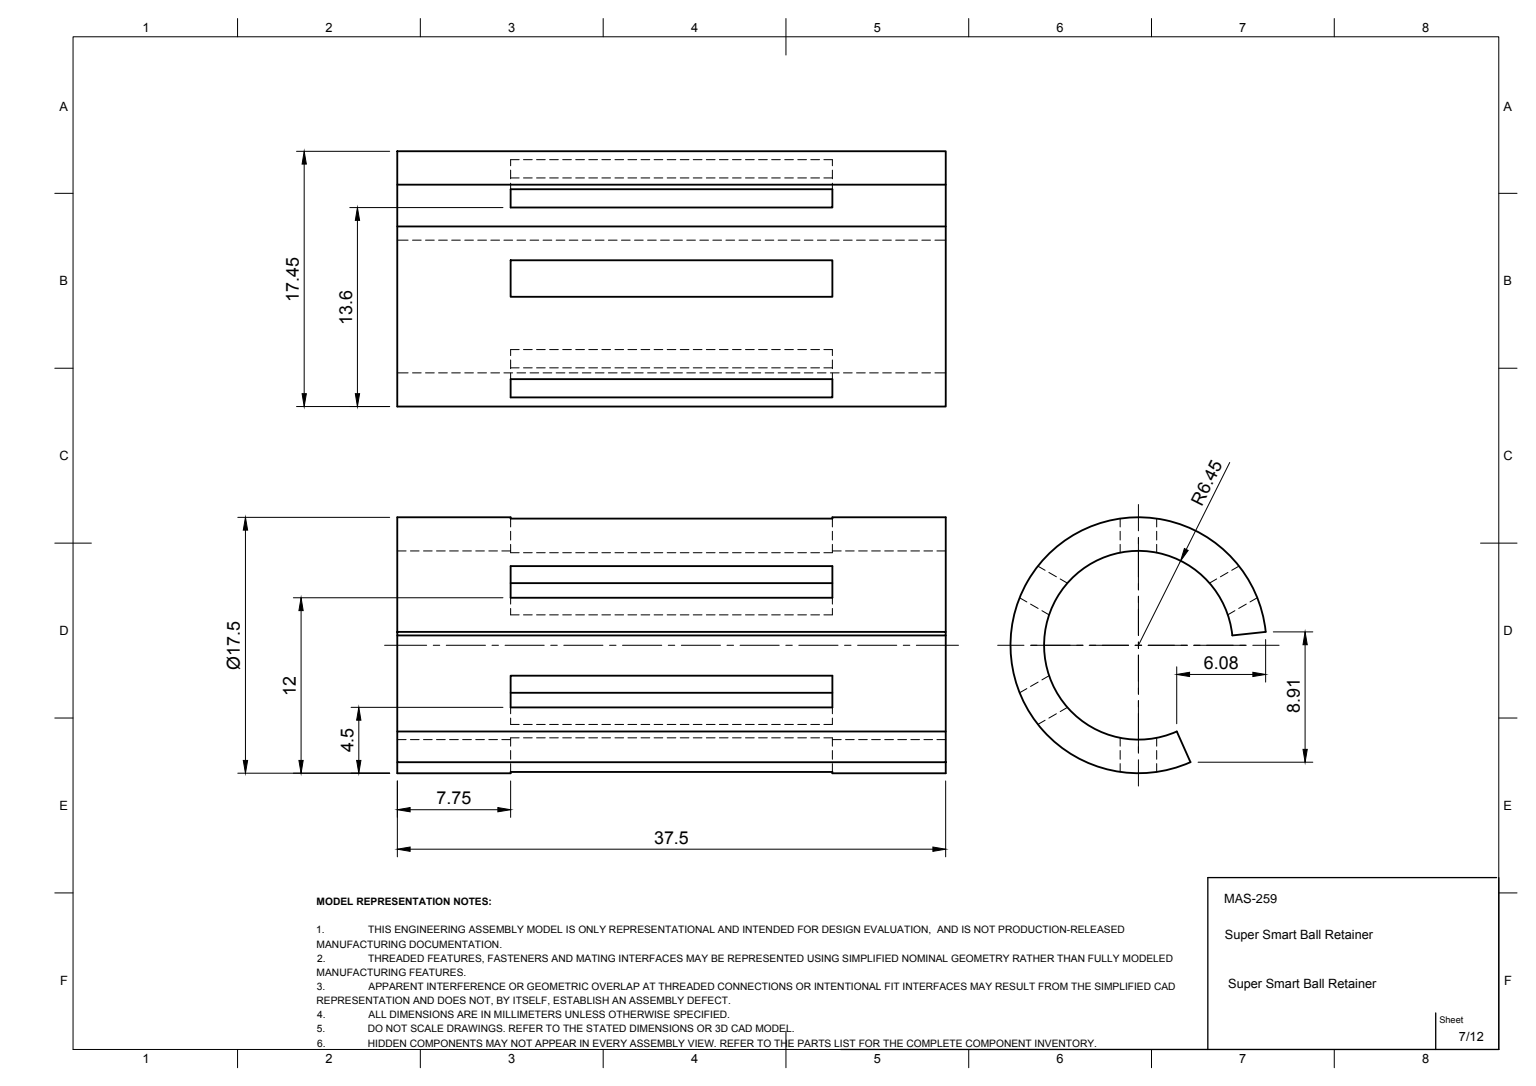
ISO-10303-21;
HEADER;
/* Generated by software containing ST-Developer
 * from STEP Tools, Inc. (www.steptools.com) 
 */

FILE_DESCRIPTION(
/* description */ (''),
/* implementation_level */ '2;1');

FILE_NAME(
/* name */ 'Super Smart Ball Retainer.step',
/* time_stamp */ '2026-10-15T13:30:17-07:00',
/* author */ (''),
/* organization */ (''),
/* preprocessor_version */ 'ST-DEVELOPER v20.2',
/* originating_system */ 'Autodesk Translation Framework v15.15.0.0',
/* authorisation */ '');

FILE_SCHEMA (('AUTOMOTIVE_DESIGN { 1 0 10303 214 3 1 1 }'));
ENDSEC;

DATA;
#10=MECHANICAL_DESIGN_GEOMETRIC_PRESENTATION_REPRESENTATION('',(#1038),#71795);
#1018=SHAPE_REPRESENTATION_RELATIONSHIP('SRR','None',#72022,#1028);
#1028=ADVANCED_BREP_SHAPE_REPRESENTATION('',(#1048),#71790);
#1038=STYLED_ITEM('',(#72081),#1048);
#1048=MANIFOLD_SOLID_BREP('Body1',#13640);
#1549=FACE_BOUND('',#2923,.T.);
#1550=FACE_BOUND('',#2924,.T.);
#1551=FACE_BOUND('',#2925,.T.);
#1552=FACE_BOUND('',#2926,.T.);
#1553=FACE_BOUND('',#2927,.T.);
#1554=FACE_BOUND('',#2929,.T.);
#1555=FACE_BOUND('',#2930,.T.);
#1556=FACE_BOUND('',#2931,.T.);
#1557=FACE_BOUND('',#2932,.T.);
#1558=FACE_BOUND('',#2933,.T.);
#1628=PLANE('',#14061);
#1629=PLANE('',#14062);
#1630=PLANE('',#14065);
#1631=PLANE('',#14066);
#1632=PLANE('',#14069);
#1633=PLANE('',#14070);
#1634=PLANE('',#14073);
#1635=PLANE('',#14074);
#1636=PLANE('',#14077);
#1637=PLANE('',#14078);
#1638=PLANE('',#14081);
#1639=PLANE('',#14082);
#1640=PLANE('',#14085);
#1641=PLANE('',#14086);
#1642=PLANE('',#14089);
#1643=PLANE('',#14090);
#1644=PLANE('',#14093);
#1645=PLANE('',#14094);
#1646=PLANE('',#14097);
#1647=PLANE('',#14098);
#1648=PLANE('',#14101);
#1649=PLANE('',#14102);
#1650=PLANE('',#14103);
#1651=PLANE('',#14110);
#2186=FACE_OUTER_BOUND('',#2899,.T.);
#2187=FACE_OUTER_BOUND('',#2900,.T.);
#2188=FACE_OUTER_BOUND('',#2901,.T.);
#2189=FACE_OUTER_BOUND('',#2902,.T.);
#2190=FACE_OUTER_BOUND('',#2903,.T.);
#2191=FACE_OUTER_BOUND('',#2904,.T.);
#2192=FACE_OUTER_BOUND('',#2905,.T.);
#2193=FACE_OUTER_BOUND('',#2906,.T.);
#2194=FACE_OUTER_BOUND('',#2907,.T.);
#2195=FACE_OUTER_BOUND('',#2908,.T.);
#2196=FACE_OUTER_BOUND('',#2909,.T.);
#2197=FACE_OUTER_BOUND('',#2910,.T.);
#2198=FACE_OUTER_BOUND('',#2911,.T.);
#2199=FACE_OUTER_BOUND('',#2912,.T.);
#2200=FACE_OUTER_BOUND('',#2913,.T.);
#2201=FACE_OUTER_BOUND('',#2914,.T.);
#2202=FACE_OUTER_BOUND('',#2915,.T.);
#2203=FACE_OUTER_BOUND('',#2916,.T.);
#2204=FACE_OUTER_BOUND('',#2917,.T.);
#2205=FACE_OUTER_BOUND('',#2918,.T.);
#2206=FACE_OUTER_BOUND('',#2919,.T.);
#2207=FACE_OUTER_BOUND('',#2920,.T.);
#2208=FACE_OUTER_BOUND('',#2921,.T.);
#2209=FACE_OUTER_BOUND('',#2922,.T.);
#2210=FACE_OUTER_BOUND('',#2928,.T.);
#2211=FACE_OUTER_BOUND('',#2934,.T.);
#2899=EDGE_LOOP('',(#9713,#9714,#9715,#9716));
#2900=EDGE_LOOP('',(#9717,#9718,#9719,#9720));
#2901=EDGE_LOOP('',(#9721,#9722,#9723,#9724));
#2902=EDGE_LOOP('',(#9725,#9726,#9727,#9728));
#2903=EDGE_LOOP('',(#9729,#9730,#9731,#9732));
#2904=EDGE_LOOP('',(#9733,#9734,#9735,#9736));
#2905=EDGE_LOOP('',(#9737,#9738,#9739,#9740));
#2906=EDGE_LOOP('',(#9741,#9742,#9743,#9744));
#2907=EDGE_LOOP('',(#9745,#9746,#9747,#9748));
#2908=EDGE_LOOP('',(#9749,#9750,#9751,#9752));
#2909=EDGE_LOOP('',(#9753,#9754,#9755,#9756));
#2910=EDGE_LOOP('',(#9757,#9758,#9759,#9760));
#2911=EDGE_LOOP('',(#9761,#9762,#9763,#9764));
#2912=EDGE_LOOP('',(#9765,#9766,#9767,#9768));
#2913=EDGE_LOOP('',(#9769,#9770,#9771,#9772));
#2914=EDGE_LOOP('',(#9773,#9774,#9775,#9776));
#2915=EDGE_LOOP('',(#9777,#9778,#9779,#9780));
#2916=EDGE_LOOP('',(#9781,#9782,#9783,#9784));
#2917=EDGE_LOOP('',(#9785,#9786,#9787,#9788));
#2918=EDGE_LOOP('',(#9789,#9790,#9791,#9792));
#2919=EDGE_LOOP('',(#9793,#9794,#9795,#9796));
#2920=EDGE_LOOP('',(#9797,#9798,#9799,#9800));
#2921=EDGE_LOOP('',(#9801,#9802,#9803,#9804));
#2922=EDGE_LOOP('',(#9805,#9806,#9807,#9808));
#2923=EDGE_LOOP('',(#9809,#9810,#9811,#9812));
#2924=EDGE_LOOP('',(#9813,#9814,#9815,#9816));
#2925=EDGE_LOOP('',(#9817,#9818,#9819,#9820));
#2926=EDGE_LOOP('',(#9821,#9822,#9823,#9824));
#2927=EDGE_LOOP('',(#9825,#9826,#9827,#9828));
#2928=EDGE_LOOP('',(#9829,#9830,#9831,#9832));
#2929=EDGE_LOOP('',(#9833,#9834,#9835,#9836));
#2930=EDGE_LOOP('',(#9837,#9838,#9839,#9840));
#2931=EDGE_LOOP('',(#9841,#9842,#9843,#9844));
#2932=EDGE_LOOP('',(#9845,#9846,#9847,#9848));
#2933=EDGE_LOOP('',(#9849,#9850,#9851,#9852));
#2934=EDGE_LOOP('',(#9853,#9854,#9855,#9856));
#3537=CIRCLE('',#14063,8.75);
#3538=CIRCLE('',#14064,6.45);
#3539=CIRCLE('',#14067,8.75);
#3540=CIRCLE('',#14068,6.45);
#3541=CIRCLE('',#14071,8.75);
#3542=CIRCLE('',#14072,6.45);
#3543=CIRCLE('',#14075,8.75);
#3544=CIRCLE('',#14076,6.45);
#3545=CIRCLE('',#14079,8.75);
#3546=CIRCLE('',#14080,6.45);
#3547=CIRCLE('',#14083,8.75);
#3548=CIRCLE('',#14084,6.45);
#3549=CIRCLE('',#14087,8.75);
#3550=CIRCLE('',#14088,6.45);
#3551=CIRCLE('',#14091,8.75);
#3552=CIRCLE('',#14092,6.45);
#3553=CIRCLE('',#14095,8.75);
#3554=CIRCLE('',#14096,6.45);
#3555=CIRCLE('',#14099,8.75);
#3556=CIRCLE('',#14100,6.45);
#3557=CIRCLE('',#14104,6.45);
#3558=CIRCLE('',#14105,8.75);
#3559=CIRCLE('',#14107,8.75);
#3560=CIRCLE('',#14109,6.45);
#4035=LINE('',#19743,#4946);
#4036=LINE('',#19745,#4947);
#4037=LINE('',#19747,#4948);
#4038=LINE('',#19748,#4949);
#4039=LINE('',#19754,#4950);
#4040=LINE('',#19757,#4951);
#4041=LINE('',#19759,#4952);
#4042=LINE('',#19760,#4953);
#4043=LINE('',#19767,#4954);
#4044=LINE('',#19769,#4955);
#4045=LINE('',#19771,#4956);
#4046=LINE('',#19772,#4957);
#4047=LINE('',#19778,#4958);
#4048=LINE('',#19781,#4959);
#4049=LINE('',#19783,#4960);
#4050=LINE('',#19784,#4961);
#4051=LINE('',#19791,#4962);
#4052=LINE('',#19793,#4963);
#4053=LINE('',#19795,#4964);
#4054=LINE('',#19796,#4965);
#4055=LINE('',#19802,#4966);
#4056=LINE('',#19805,#4967);
#4057=LINE('',#19807,#4968);
#4058=LINE('',#19808,#4969);
#4059=LINE('',#19815,#4970);
#4060=LINE('',#19817,#4971);
#4061=LINE('',#19819,#4972);
#4062=LINE('',#19820,#4973);
#4063=LINE('',#19826,#4974);
#4064=LINE('',#19829,#4975);
#4065=LINE('',#19831,#4976);
#4066=LINE('',#19832,#4977);
#4067=LINE('',#19839,#4978);
#4068=LINE('',#19841,#4979);
#4069=LINE('',#19843,#4980);
#4070=LINE('',#19844,#4981);
#4071=LINE('',#19850,#4982);
#4072=LINE('',#19853,#4983);
#4073=LINE('',#19855,#4984);
#4074=LINE('',#19856,#4985);
#4075=LINE('',#19863,#4986);
#4076=LINE('',#19865,#4987);
#4077=LINE('',#19867,#4988);
#4078=LINE('',#19868,#4989);
#4079=LINE('',#19872,#4990);
#4080=LINE('',#19874,#4991);
#4081=LINE('',#19876,#4992);
#4082=LINE('',#19877,#4993);
#4946=VECTOR('',#15852,10.);
#4947=VECTOR('',#15853,10.);
#4948=VECTOR('',#15854,10.);
#4949=VECTOR('',#15855,10.);
#4950=VECTOR('',#15862,10.);
#4951=VECTOR('',#15865,10.);
#4952=VECTOR('',#15866,10.);
#4953=VECTOR('',#15867,10.);
#4954=VECTOR('',#15876,10.);
#4955=VECTOR('',#15877,10.);
#4956=VECTOR('',#15878,10.);
#4957=VECTOR('',#15879,10.);
#4958=VECTOR('',#15886,10.);
#4959=VECTOR('',#15889,10.);
#4960=VECTOR('',#15890,10.);
#4961=VECTOR('',#15891,10.);
#4962=VECTOR('',#15900,10.);
#4963=VECTOR('',#15901,10.);
#4964=VECTOR('',#15902,10.);
#4965=VECTOR('',#15903,10.);
#4966=VECTOR('',#15910,9.99999999999999);
#4967=VECTOR('',#15913,10.);
#4968=VECTOR('',#15914,10.);
#4969=VECTOR('',#15915,9.99999999999999);
#4970=VECTOR('',#15924,10.);
#4971=VECTOR('',#15925,9.99999999999999);
#4972=VECTOR('',#15926,10.);
#4973=VECTOR('',#15927,9.99999999999999);
#4974=VECTOR('',#15934,10.);
#4975=VECTOR('',#15937,10.);
#4976=VECTOR('',#15938,10.);
#4977=VECTOR('',#15939,10.);
#4978=VECTOR('',#15948,10.);
#4979=VECTOR('',#15949,9.99999999999999);
#4980=VECTOR('',#15950,10.);
#4981=VECTOR('',#15951,9.99999999999999);
#4982=VECTOR('',#15958,10.);
#4983=VECTOR('',#15961,10.);
#4984=VECTOR('',#15962,10.);
#4985=VECTOR('',#15963,10.);
#4986=VECTOR('',#15972,10.);
#4987=VECTOR('',#15973,10.);
#4988=VECTOR('',#15974,10.);
#4989=VECTOR('',#15975,10.);
#4990=VECTOR('',#15978,10.);
#4991=VECTOR('',#15979,10.);
#4992=VECTOR('',#15980,10.);
#4993=VECTOR('',#15981,10.);
#5916=VERTEX_POINT('',#19741);
#5917=VERTEX_POINT('',#19742);
#5918=VERTEX_POINT('',#19744);
#5919=VERTEX_POINT('',#19746);
#5920=VERTEX_POINT('',#19750);
#5921=VERTEX_POINT('',#19752);
#5922=VERTEX_POINT('',#19756);
#5923=VERTEX_POINT('',#19758);
#5924=VERTEX_POINT('',#19765);
#5925=VERTEX_POINT('',#19766);
#5926=VERTEX_POINT('',#19768);
#5927=VERTEX_POINT('',#19770);
#5928=VERTEX_POINT('',#19774);
#5929=VERTEX_POINT('',#19776);
#5930=VERTEX_POINT('',#19780);
#5931=VERTEX_POINT('',#19782);
#5932=VERTEX_POINT('',#19789);
#5933=VERTEX_POINT('',#19790);
#5934=VERTEX_POINT('',#19792);
#5935=VERTEX_POINT('',#19794);
#5936=VERTEX_POINT('',#19798);
#5937=VERTEX_POINT('',#19800);
#5938=VERTEX_POINT('',#19804);
#5939=VERTEX_POINT('',#19806);
#5940=VERTEX_POINT('',#19813);
#5941=VERTEX_POINT('',#19814);
#5942=VERTEX_POINT('',#19816);
#5943=VERTEX_POINT('',#19818);
#5944=VERTEX_POINT('',#19822);
#5945=VERTEX_POINT('',#19824);
#5946=VERTEX_POINT('',#19828);
#5947=VERTEX_POINT('',#19830);
#5948=VERTEX_POINT('',#19837);
#5949=VERTEX_POINT('',#19838);
#5950=VERTEX_POINT('',#19840);
#5951=VERTEX_POINT('',#19842);
#5952=VERTEX_POINT('',#19846);
#5953=VERTEX_POINT('',#19848);
#5954=VERTEX_POINT('',#19852);
#5955=VERTEX_POINT('',#19854);
#5956=VERTEX_POINT('',#19861);
#5957=VERTEX_POINT('',#19862);
#5958=VERTEX_POINT('',#19864);
#5959=VERTEX_POINT('',#19866);
#5960=VERTEX_POINT('',#19870);
#5961=VERTEX_POINT('',#19871);
#5962=VERTEX_POINT('',#19873);
#5963=VERTEX_POINT('',#19875);
#7391=EDGE_CURVE('',#5916,#5917,#4035,.T.);
#7392=EDGE_CURVE('',#5916,#5918,#4036,.T.);
#7393=EDGE_CURVE('',#5919,#5918,#4037,.T.);
#7394=EDGE_CURVE('',#5919,#5917,#4038,.T.);
#7395=EDGE_CURVE('',#5917,#5920,#3537,.T.);
#7396=EDGE_CURVE('',#5921,#5919,#3538,.T.);
#7397=EDGE_CURVE('',#5920,#5921,#4039,.T.);
#7398=EDGE_CURVE('',#5920,#5922,#4040,.T.);
#7399=EDGE_CURVE('',#5923,#5921,#4041,.T.);
#7400=EDGE_CURVE('',#5923,#5922,#4042,.T.);
#7401=EDGE_CURVE('',#5922,#5916,#3539,.T.);
#7402=EDGE_CURVE('',#5918,#5923,#3540,.T.);
#7403=EDGE_CURVE('',#5924,#5925,#4043,.T.);
#7404=EDGE_CURVE('',#5924,#5926,#4044,.T.);
#7405=EDGE_CURVE('',#5927,#5926,#4045,.T.);
#7406=EDGE_CURVE('',#5927,#5925,#4046,.T.);
#7407=EDGE_CURVE('',#5925,#5928,#3541,.T.);
#7408=EDGE_CURVE('',#5929,#5927,#3542,.T.);
#7409=EDGE_CURVE('',#5928,#5929,#4047,.T.);
#7410=EDGE_CURVE('',#5928,#5930,#4048,.T.);
#7411=EDGE_CURVE('',#5931,#5929,#4049,.T.);
#7412=EDGE_CURVE('',#5931,#5930,#4050,.T.);
#7413=EDGE_CURVE('',#5930,#5924,#3543,.T.);
#7414=EDGE_CURVE('',#5926,#5931,#3544,.T.);
#7415=EDGE_CURVE('',#5932,#5933,#4051,.T.);
#7416=EDGE_CURVE('',#5932,#5934,#4052,.T.);
#7417=EDGE_CURVE('',#5935,#5934,#4053,.T.);
#7418=EDGE_CURVE('',#5935,#5933,#4054,.T.);
#7419=EDGE_CURVE('',#5933,#5936,#3545,.T.);
#7420=EDGE_CURVE('',#5937,#5935,#3546,.T.);
#7421=EDGE_CURVE('',#5936,#5937,#4055,.T.);
#7422=EDGE_CURVE('',#5936,#5938,#4056,.T.);
#7423=EDGE_CURVE('',#5939,#5937,#4057,.T.);
#7424=EDGE_CURVE('',#5939,#5938,#4058,.T.);
#7425=EDGE_CURVE('',#5938,#5932,#3547,.T.);
#7426=EDGE_CURVE('',#5934,#5939,#3548,.T.);
#7427=EDGE_CURVE('',#5940,#5941,#4059,.T.);
#7428=EDGE_CURVE('',#5940,#5942,#4060,.T.);
#7429=EDGE_CURVE('',#5943,#5942,#4061,.T.);
#7430=EDGE_CURVE('',#5943,#5941,#4062,.T.);
#7431=EDGE_CURVE('',#5941,#5944,#3549,.T.);
#7432=EDGE_CURVE('',#5945,#5943,#3550,.T.);
#7433=EDGE_CURVE('',#5944,#5945,#4063,.T.);
#7434=EDGE_CURVE('',#5944,#5946,#4064,.T.);
#7435=EDGE_CURVE('',#5947,#5945,#4065,.T.);
#7436=EDGE_CURVE('',#5947,#5946,#4066,.T.);
#7437=EDGE_CURVE('',#5946,#5940,#3551,.T.);
#7438=EDGE_CURVE('',#5942,#5947,#3552,.T.);
#7439=EDGE_CURVE('',#5948,#5949,#4067,.T.);
#7440=EDGE_CURVE('',#5948,#5950,#4068,.T.);
#7441=EDGE_CURVE('',#5951,#5950,#4069,.T.);
#7442=EDGE_CURVE('',#5951,#5949,#4070,.T.);
#7443=EDGE_CURVE('',#5949,#5952,#3553,.T.);
#7444=EDGE_CURVE('',#5953,#5951,#3554,.T.);
#7445=EDGE_CURVE('',#5952,#5953,#4071,.T.);
#7446=EDGE_CURVE('',#5952,#5954,#4072,.T.);
#7447=EDGE_CURVE('',#5955,#5953,#4073,.T.);
#7448=EDGE_CURVE('',#5955,#5954,#4074,.T.);
#7449=EDGE_CURVE('',#5954,#5948,#3555,.T.);
#7450=EDGE_CURVE('',#5950,#5955,#3556,.T.);
#7451=EDGE_CURVE('',#5956,#5957,#4075,.T.);
#7452=EDGE_CURVE('',#5958,#5956,#4076,.T.);
#7453=EDGE_CURVE('',#5959,#5958,#4077,.T.);
#7454=EDGE_CURVE('',#5957,#5959,#4078,.T.);
#7455=EDGE_CURVE('',#5960,#5961,#4079,.T.);
#7456=EDGE_CURVE('',#5962,#5960,#4080,.T.);
#7457=EDGE_CURVE('',#5963,#5962,#4081,.T.);
#7458=EDGE_CURVE('',#5961,#5963,#4082,.T.);
#7459=EDGE_CURVE('',#5961,#5956,#3557,.T.);
#7460=EDGE_CURVE('',#5963,#5958,#3558,.T.);
#7461=EDGE_CURVE('',#5962,#5959,#3559,.T.);
#7462=EDGE_CURVE('',#5960,#5957,#3560,.T.);
#9713=ORIENTED_EDGE('',*,*,#7391,.F.);
#9714=ORIENTED_EDGE('',*,*,#7392,.T.);
#9715=ORIENTED_EDGE('',*,*,#7393,.F.);
#9716=ORIENTED_EDGE('',*,*,#7394,.T.);
#9717=ORIENTED_EDGE('',*,*,#7395,.F.);
#9718=ORIENTED_EDGE('',*,*,#7394,.F.);
#9719=ORIENTED_EDGE('',*,*,#7396,.F.);
#9720=ORIENTED_EDGE('',*,*,#7397,.F.);
#9721=ORIENTED_EDGE('',*,*,#7398,.F.);
#9722=ORIENTED_EDGE('',*,*,#7397,.T.);
#9723=ORIENTED_EDGE('',*,*,#7399,.F.);
#9724=ORIENTED_EDGE('',*,*,#7400,.T.);
#9725=ORIENTED_EDGE('',*,*,#7401,.F.);
#9726=ORIENTED_EDGE('',*,*,#7400,.F.);
#9727=ORIENTED_EDGE('',*,*,#7402,.F.);
#9728=ORIENTED_EDGE('',*,*,#7392,.F.);
#9729=ORIENTED_EDGE('',*,*,#7403,.F.);
#9730=ORIENTED_EDGE('',*,*,#7404,.T.);
#9731=ORIENTED_EDGE('',*,*,#7405,.F.);
#9732=ORIENTED_EDGE('',*,*,#7406,.T.);
#9733=ORIENTED_EDGE('',*,*,#7407,.F.);
#9734=ORIENTED_EDGE('',*,*,#7406,.F.);
#9735=ORIENTED_EDGE('',*,*,#7408,.F.);
#9736=ORIENTED_EDGE('',*,*,#7409,.F.);
#9737=ORIENTED_EDGE('',*,*,#7410,.F.);
#9738=ORIENTED_EDGE('',*,*,#7409,.T.);
#9739=ORIENTED_EDGE('',*,*,#7411,.F.);
#9740=ORIENTED_EDGE('',*,*,#7412,.T.);
#9741=ORIENTED_EDGE('',*,*,#7413,.F.);
#9742=ORIENTED_EDGE('',*,*,#7412,.F.);
#9743=ORIENTED_EDGE('',*,*,#7414,.F.);
#9744=ORIENTED_EDGE('',*,*,#7404,.F.);
#9745=ORIENTED_EDGE('',*,*,#7415,.F.);
#9746=ORIENTED_EDGE('',*,*,#7416,.T.);
#9747=ORIENTED_EDGE('',*,*,#7417,.F.);
#9748=ORIENTED_EDGE('',*,*,#7418,.T.);
#9749=ORIENTED_EDGE('',*,*,#7419,.F.);
#9750=ORIENTED_EDGE('',*,*,#7418,.F.);
#9751=ORIENTED_EDGE('',*,*,#7420,.F.);
#9752=ORIENTED_EDGE('',*,*,#7421,.F.);
#9753=ORIENTED_EDGE('',*,*,#7422,.F.);
#9754=ORIENTED_EDGE('',*,*,#7421,.T.);
#9755=ORIENTED_EDGE('',*,*,#7423,.F.);
#9756=ORIENTED_EDGE('',*,*,#7424,.T.);
#9757=ORIENTED_EDGE('',*,*,#7425,.F.);
#9758=ORIENTED_EDGE('',*,*,#7424,.F.);
#9759=ORIENTED_EDGE('',*,*,#7426,.F.);
#9760=ORIENTED_EDGE('',*,*,#7416,.F.);
#9761=ORIENTED_EDGE('',*,*,#7427,.F.);
#9762=ORIENTED_EDGE('',*,*,#7428,.T.);
#9763=ORIENTED_EDGE('',*,*,#7429,.F.);
#9764=ORIENTED_EDGE('',*,*,#7430,.T.);
#9765=ORIENTED_EDGE('',*,*,#7431,.F.);
#9766=ORIENTED_EDGE('',*,*,#7430,.F.);
#9767=ORIENTED_EDGE('',*,*,#7432,.F.);
#9768=ORIENTED_EDGE('',*,*,#7433,.F.);
#9769=ORIENTED_EDGE('',*,*,#7434,.F.);
#9770=ORIENTED_EDGE('',*,*,#7433,.T.);
#9771=ORIENTED_EDGE('',*,*,#7435,.F.);
#9772=ORIENTED_EDGE('',*,*,#7436,.T.);
#9773=ORIENTED_EDGE('',*,*,#7437,.F.);
#9774=ORIENTED_EDGE('',*,*,#7436,.F.);
#9775=ORIENTED_EDGE('',*,*,#7438,.F.);
#9776=ORIENTED_EDGE('',*,*,#7428,.F.);
#9777=ORIENTED_EDGE('',*,*,#7439,.F.);
#9778=ORIENTED_EDGE('',*,*,#7440,.T.);
#9779=ORIENTED_EDGE('',*,*,#7441,.F.);
#9780=ORIENTED_EDGE('',*,*,#7442,.T.);
#9781=ORIENTED_EDGE('',*,*,#7443,.F.);
#9782=ORIENTED_EDGE('',*,*,#7442,.F.);
#9783=ORIENTED_EDGE('',*,*,#7444,.F.);
#9784=ORIENTED_EDGE('',*,*,#7445,.F.);
#9785=ORIENTED_EDGE('',*,*,#7446,.F.);
#9786=ORIENTED_EDGE('',*,*,#7445,.T.);
#9787=ORIENTED_EDGE('',*,*,#7447,.F.);
#9788=ORIENTED_EDGE('',*,*,#7448,.T.);
#9789=ORIENTED_EDGE('',*,*,#7449,.F.);
#9790=ORIENTED_EDGE('',*,*,#7448,.F.);
#9791=ORIENTED_EDGE('',*,*,#7450,.F.);
#9792=ORIENTED_EDGE('',*,*,#7440,.F.);
#9793=ORIENTED_EDGE('',*,*,#7451,.F.);
#9794=ORIENTED_EDGE('',*,*,#7452,.F.);
#9795=ORIENTED_EDGE('',*,*,#7453,.F.);
#9796=ORIENTED_EDGE('',*,*,#7454,.F.);
#9797=ORIENTED_EDGE('',*,*,#7455,.F.);
#9798=ORIENTED_EDGE('',*,*,#7456,.F.);
#9799=ORIENTED_EDGE('',*,*,#7457,.F.);
#9800=ORIENTED_EDGE('',*,*,#7458,.F.);
#9801=ORIENTED_EDGE('',*,*,#7452,.T.);
#9802=ORIENTED_EDGE('',*,*,#7459,.F.);
#9803=ORIENTED_EDGE('',*,*,#7458,.T.);
#9804=ORIENTED_EDGE('',*,*,#7460,.T.);
#9805=ORIENTED_EDGE('',*,*,#7453,.T.);
#9806=ORIENTED_EDGE('',*,*,#7460,.F.);
#9807=ORIENTED_EDGE('',*,*,#7457,.T.);
#9808=ORIENTED_EDGE('',*,*,#7461,.T.);
#9809=ORIENTED_EDGE('',*,*,#7398,.T.);
#9810=ORIENTED_EDGE('',*,*,#7401,.T.);
#9811=ORIENTED_EDGE('',*,*,#7391,.T.);
#9812=ORIENTED_EDGE('',*,*,#7395,.T.);
#9813=ORIENTED_EDGE('',*,*,#7410,.T.);
#9814=ORIENTED_EDGE('',*,*,#7413,.T.);
#9815=ORIENTED_EDGE('',*,*,#7403,.T.);
#9816=ORIENTED_EDGE('',*,*,#7407,.T.);
#9817=ORIENTED_EDGE('',*,*,#7422,.T.);
#9818=ORIENTED_EDGE('',*,*,#7425,.T.);
#9819=ORIENTED_EDGE('',*,*,#7415,.T.);
#9820=ORIENTED_EDGE('',*,*,#7419,.T.);
#9821=ORIENTED_EDGE('',*,*,#7434,.T.);
#9822=ORIENTED_EDGE('',*,*,#7437,.T.);
#9823=ORIENTED_EDGE('',*,*,#7427,.T.);
#9824=ORIENTED_EDGE('',*,*,#7431,.T.);
#9825=ORIENTED_EDGE('',*,*,#7446,.T.);
#9826=ORIENTED_EDGE('',*,*,#7449,.T.);
#9827=ORIENTED_EDGE('',*,*,#7439,.T.);
#9828=ORIENTED_EDGE('',*,*,#7443,.T.);
#9829=ORIENTED_EDGE('',*,*,#7451,.T.);
#9830=ORIENTED_EDGE('',*,*,#7462,.F.);
#9831=ORIENTED_EDGE('',*,*,#7455,.T.);
#9832=ORIENTED_EDGE('',*,*,#7459,.T.);
#9833=ORIENTED_EDGE('',*,*,#7399,.T.);
#9834=ORIENTED_EDGE('',*,*,#7396,.T.);
#9835=ORIENTED_EDGE('',*,*,#7393,.T.);
#9836=ORIENTED_EDGE('',*,*,#7402,.T.);
#9837=ORIENTED_EDGE('',*,*,#7411,.T.);
#9838=ORIENTED_EDGE('',*,*,#7408,.T.);
#9839=ORIENTED_EDGE('',*,*,#7405,.T.);
#9840=ORIENTED_EDGE('',*,*,#7414,.T.);
#9841=ORIENTED_EDGE('',*,*,#7423,.T.);
#9842=ORIENTED_EDGE('',*,*,#7420,.T.);
#9843=ORIENTED_EDGE('',*,*,#7417,.T.);
#9844=ORIENTED_EDGE('',*,*,#7426,.T.);
#9845=ORIENTED_EDGE('',*,*,#7435,.T.);
#9846=ORIENTED_EDGE('',*,*,#7432,.T.);
#9847=ORIENTED_EDGE('',*,*,#7429,.T.);
#9848=ORIENTED_EDGE('',*,*,#7438,.T.);
#9849=ORIENTED_EDGE('',*,*,#7447,.T.);
#9850=ORIENTED_EDGE('',*,*,#7444,.T.);
#9851=ORIENTED_EDGE('',*,*,#7441,.T.);
#9852=ORIENTED_EDGE('',*,*,#7450,.T.);
#9853=ORIENTED_EDGE('',*,*,#7454,.T.);
#9854=ORIENTED_EDGE('',*,*,#7461,.F.);
#9855=ORIENTED_EDGE('',*,*,#7456,.T.);
#9856=ORIENTED_EDGE('',*,*,#7462,.T.);
#12916=CYLINDRICAL_SURFACE('',#14106,8.75);
#12917=CYLINDRICAL_SURFACE('',#14108,6.45);
#13146=ADVANCED_FACE('',(#2186),#1628,.F.);
#13147=ADVANCED_FACE('',(#2187),#1629,.T.);
#13148=ADVANCED_FACE('',(#2188),#1630,.F.);
#13149=ADVANCED_FACE('',(#2189),#1631,.F.);
#13150=ADVANCED_FACE('',(#2190),#1632,.F.);
#13151=ADVANCED_FACE('',(#2191),#1633,.T.);
#13152=ADVANCED_FACE('',(#2192),#1634,.F.);
#13153=ADVANCED_FACE('',(#2193),#1635,.F.);
#13154=ADVANCED_FACE('',(#2194),#1636,.F.);
#13155=ADVANCED_FACE('',(#2195),#1637,.T.);
#13156=ADVANCED_FACE('',(#2196),#1638,.F.);
#13157=ADVANCED_FACE('',(#2197),#1639,.F.);
#13158=ADVANCED_FACE('',(#2198),#1640,.F.);
#13159=ADVANCED_FACE('',(#2199),#1641,.T.);
#13160=ADVANCED_FACE('',(#2200),#1642,.F.);
#13161=ADVANCED_FACE('',(#2201),#1643,.F.);
#13162=ADVANCED_FACE('',(#2202),#1644,.F.);
#13163=ADVANCED_FACE('',(#2203),#1645,.T.);
#13164=ADVANCED_FACE('',(#2204),#1646,.F.);
#13165=ADVANCED_FACE('',(#2205),#1647,.F.);
#13166=ADVANCED_FACE('',(#2206),#1648,.F.);
#13167=ADVANCED_FACE('',(#2207),#1649,.F.);
#13168=ADVANCED_FACE('',(#2208),#1650,.T.);
#13169=ADVANCED_FACE('',(#2209,#1549,#1550,#1551,#1552,#1553),#12916,.T.);
#13170=ADVANCED_FACE('',(#2210,#1554,#1555,#1556,#1557,#1558),#12917,.F.);
#13171=ADVANCED_FACE('',(#2211),#1651,.T.);
#13640=CLOSED_SHELL('',(#13146,#13147,#13148,#13149,#13150,#13151,#13152,
#13153,#13154,#13155,#13156,#13157,#13158,#13159,#13160,#13161,#13162,#13163,
#13164,#13165,#13166,#13167,#13168,#13169,#13170,#13171));
#14060=AXIS2_PLACEMENT_3D('',#19739,#15848,#15849);
#14061=AXIS2_PLACEMENT_3D('',#19740,#15850,#15851);
#14062=AXIS2_PLACEMENT_3D('',#19749,#15856,#15857);
#14063=AXIS2_PLACEMENT_3D('',#19751,#15858,#15859);
#14064=AXIS2_PLACEMENT_3D('',#19753,#15860,#15861);
#14065=AXIS2_PLACEMENT_3D('',#19755,#15863,#15864);
#14066=AXIS2_PLACEMENT_3D('',#19761,#15868,#15869);
#14067=AXIS2_PLACEMENT_3D('',#19762,#15870,#15871);
#14068=AXIS2_PLACEMENT_3D('',#19763,#15872,#15873);
#14069=AXIS2_PLACEMENT_3D('',#19764,#15874,#15875);
#14070=AXIS2_PLACEMENT_3D('',#19773,#15880,#15881);
#14071=AXIS2_PLACEMENT_3D('',#19775,#15882,#15883);
#14072=AXIS2_PLACEMENT_3D('',#19777,#15884,#15885);
#14073=AXIS2_PLACEMENT_3D('',#19779,#15887,#15888);
#14074=AXIS2_PLACEMENT_3D('',#19785,#15892,#15893);
#14075=AXIS2_PLACEMENT_3D('',#19786,#15894,#15895);
#14076=AXIS2_PLACEMENT_3D('',#19787,#15896,#15897);
#14077=AXIS2_PLACEMENT_3D('',#19788,#15898,#15899);
#14078=AXIS2_PLACEMENT_3D('',#19797,#15904,#15905);
#14079=AXIS2_PLACEMENT_3D('',#19799,#15906,#15907);
#14080=AXIS2_PLACEMENT_3D('',#19801,#15908,#15909);
#14081=AXIS2_PLACEMENT_3D('',#19803,#15911,#15912);
#14082=AXIS2_PLACEMENT_3D('',#19809,#15916,#15917);
#14083=AXIS2_PLACEMENT_3D('',#19810,#15918,#15919);
#14084=AXIS2_PLACEMENT_3D('',#19811,#15920,#15921);
#14085=AXIS2_PLACEMENT_3D('',#19812,#15922,#15923);
#14086=AXIS2_PLACEMENT_3D('',#19821,#15928,#15929);
#14087=AXIS2_PLACEMENT_3D('',#19823,#15930,#15931);
#14088=AXIS2_PLACEMENT_3D('',#19825,#15932,#15933);
#14089=AXIS2_PLACEMENT_3D('',#19827,#15935,#15936);
#14090=AXIS2_PLACEMENT_3D('',#19833,#15940,#15941);
#14091=AXIS2_PLACEMENT_3D('',#19834,#15942,#15943);
#14092=AXIS2_PLACEMENT_3D('',#19835,#15944,#15945);
#14093=AXIS2_PLACEMENT_3D('',#19836,#15946,#15947);
#14094=AXIS2_PLACEMENT_3D('',#19845,#15952,#15953);
#14095=AXIS2_PLACEMENT_3D('',#19847,#15954,#15955);
#14096=AXIS2_PLACEMENT_3D('',#19849,#15956,#15957);
#14097=AXIS2_PLACEMENT_3D('',#19851,#15959,#15960);
#14098=AXIS2_PLACEMENT_3D('',#19857,#15964,#15965);
#14099=AXIS2_PLACEMENT_3D('',#19858,#15966,#15967);
#14100=AXIS2_PLACEMENT_3D('',#19859,#15968,#15969);
#14101=AXIS2_PLACEMENT_3D('',#19860,#15970,#15971);
#14102=AXIS2_PLACEMENT_3D('',#19869,#15976,#15977);
#14103=AXIS2_PLACEMENT_3D('',#19878,#15982,#15983);
#14104=AXIS2_PLACEMENT_3D('',#19879,#15984,#15985);
#14105=AXIS2_PLACEMENT_3D('',#19880,#15986,#15987);
#14106=AXIS2_PLACEMENT_3D('',#19881,#15988,#15989);
#14107=AXIS2_PLACEMENT_3D('',#19882,#15990,#15991);
#14108=AXIS2_PLACEMENT_3D('',#19883,#15992,#15993);
#14109=AXIS2_PLACEMENT_3D('',#19884,#15994,#15995);
#14110=AXIS2_PLACEMENT_3D('',#19885,#15996,#15997);
#15848=DIRECTION('axis',(0.,0.,1.));
#15849=DIRECTION('refdir',(1.,0.,0.));
#15850=DIRECTION('center_axis',(0.,0.258819045102523,0.965925826289068));
#15851=DIRECTION('ref_axis',(0.,-0.965925826289068,0.258819045102523));
#15852=DIRECTION('',(-1.,0.,0.));
#15853=DIRECTION('',(0.,-0.965925826289068,0.258819045102523));
#15854=DIRECTION('',(1.,0.,0.));
#15855=DIRECTION('',(0.,0.965925826289068,-0.258819045102523));
#15856=DIRECTION('center_axis',(1.,0.,0.));
#15857=DIRECTION('ref_axis',(0.,0.,-1.));
#15858=DIRECTION('center_axis',(-1.,0.,0.));
#15859=DIRECTION('ref_axis',(0.,1.,0.));
#15860=DIRECTION('center_axis',(1.,0.,0.));
#15861=DIRECTION('ref_axis',(0.,1.,0.));
#15862=DIRECTION('',(0.,-0.965925826289068,0.258819045102523));
#15863=DIRECTION('center_axis',(0.,-0.258819045102523,-0.965925826289068));
#15864=DIRECTION('ref_axis',(0.,0.965925826289068,-0.258819045102523));
#15865=DIRECTION('',(1.,0.,0.));
#15866=DIRECTION('',(-1.,0.,0.));
#15867=DIRECTION('',(0.,0.965925826289068,-0.258819045102523));
#15868=DIRECTION('center_axis',(1.,0.,0.));
#15869=DIRECTION('ref_axis',(0.,0.,-1.));
#15870=DIRECTION('center_axis',(1.,0.,0.));
#15871=DIRECTION('ref_axis',(0.,1.,0.));
#15872=DIRECTION('center_axis',(-1.,0.,0.));
#15873=DIRECTION('ref_axis',(0.,1.,0.));
#15874=DIRECTION('center_axis',(0.,-0.707106781186549,0.707106781186546));
#15875=DIRECTION('ref_axis',(0.,-0.707106781186546,-0.707106781186549));
#15876=DIRECTION('',(-1.,0.,0.));
#15877=DIRECTION('',(0.,-0.707106781186546,-0.707106781186549));
#15878=DIRECTION('',(1.,0.,0.));
#15879=DIRECTION('',(0.,0.707106781186546,0.707106781186549));
#15880=DIRECTION('center_axis',(1.,0.,0.));
#15881=DIRECTION('ref_axis',(0.,0.,-1.));
#15882=DIRECTION('center_axis',(-1.,0.,0.));
#15883=DIRECTION('ref_axis',(0.,1.,0.));
#15884=DIRECTION('center_axis',(1.,0.,0.));
#15885=DIRECTION('ref_axis',(0.,1.,0.));
#15886=DIRECTION('',(0.,-0.707106781186547,-0.707106781186547));
#15887=DIRECTION('center_axis',(0.,0.707106781186548,-0.707106781186548));
#15888=DIRECTION('ref_axis',(0.,0.707106781186548,0.707106781186548));
#15889=DIRECTION('',(1.,0.,0.));
#15890=DIRECTION('',(-1.,0.,0.));
#15891=DIRECTION('',(0.,0.707106781186547,0.707106781186547));
#15892=DIRECTION('center_axis',(1.,0.,0.));
#15893=DIRECTION('ref_axis',(0.,0.,-1.));
#15894=DIRECTION('center_axis',(1.,0.,0.));
#15895=DIRECTION('ref_axis',(0.,1.,0.));
#15896=DIRECTION('center_axis',(-1.,0.,0.));
#15897=DIRECTION('ref_axis',(0.,1.,0.));
#15898=DIRECTION('center_axis',(0.,-0.965925826289068,-0.258819045102522));
#15899=DIRECTION('ref_axis',(0.,0.258819045102522,-0.965925826289068));
#15900=DIRECTION('',(-1.,0.,0.));
#15901=DIRECTION('',(0.,0.258819045102522,-0.965925826289068));
#15902=DIRECTION('',(1.,0.,0.));
#15903=DIRECTION('',(0.,-0.258819045102522,0.965925826289068));
#15904=DIRECTION('center_axis',(1.,0.,0.));
#15905=DIRECTION('ref_axis',(0.,0.,-1.));
#15906=DIRECTION('center_axis',(-1.,0.,0.));
#15907=DIRECTION('ref_axis',(0.,1.,0.));
#15908=DIRECTION('center_axis',(1.,0.,0.));
#15909=DIRECTION('ref_axis',(0.,1.,0.));
#15910=DIRECTION('',(0.,0.25881904510252,-0.965925826289068));
#15911=DIRECTION('center_axis',(0.,0.965925826289069,0.25881904510252));
#15912=DIRECTION('ref_axis',(0.,-0.25881904510252,0.965925826289069));
#15913=DIRECTION('',(1.,0.,0.));
#15914=DIRECTION('',(-1.,0.,0.));
#15915=DIRECTION('',(0.,-0.25881904510252,0.965925826289068));
#15916=DIRECTION('center_axis',(1.,0.,0.));
#15917=DIRECTION('ref_axis',(0.,0.,-1.));
#15918=DIRECTION('center_axis',(1.,0.,0.));
#15919=DIRECTION('ref_axis',(0.,1.,0.));
#15920=DIRECTION('center_axis',(-1.,0.,0.));
#15921=DIRECTION('ref_axis',(0.,1.,0.));
#15922=DIRECTION('center_axis',(0.,-0.25881904510252,-0.965925826289069));
#15923=DIRECTION('ref_axis',(0.,0.965925826289069,-0.25881904510252));
#15924=DIRECTION('',(-1.,0.,0.));
#15925=DIRECTION('',(0.,0.965925826289068,-0.25881904510252));
#15926=DIRECTION('',(1.,0.,0.));
#15927=DIRECTION('',(0.,-0.965925826289068,0.25881904510252));
#15928=DIRECTION('center_axis',(1.,0.,0.));
#15929=DIRECTION('ref_axis',(0.,0.,-1.));
#15930=DIRECTION('center_axis',(-1.,0.,0.));
#15931=DIRECTION('ref_axis',(0.,1.,0.));
#15932=DIRECTION('center_axis',(1.,0.,0.));
#15933=DIRECTION('ref_axis',(0.,1.,0.));
#15934=DIRECTION('',(0.,0.965925826289069,-0.25881904510252));
#15935=DIRECTION('center_axis',(0.,0.25881904510252,0.965925826289069));
#15936=DIRECTION('ref_axis',(0.,-0.965925826289069,0.25881904510252));
#15937=DIRECTION('',(1.,0.,0.));
#15938=DIRECTION('',(-1.,0.,0.));
#15939=DIRECTION('',(0.,-0.965925826289069,0.25881904510252));
#15940=DIRECTION('center_axis',(1.,0.,0.));
#15941=DIRECTION('ref_axis',(0.,0.,-1.));
#15942=DIRECTION('center_axis',(1.,0.,0.));
#15943=DIRECTION('ref_axis',(0.,1.,0.));
#15944=DIRECTION('center_axis',(-1.,0.,0.));
#15945=DIRECTION('ref_axis',(0.,1.,0.));
#15946=DIRECTION('center_axis',(0.,0.965925826289069,0.25881904510252));
#15947=DIRECTION('ref_axis',(0.,-0.25881904510252,0.965925826289069));
#15948=DIRECTION('',(-1.,0.,0.));
#15949=DIRECTION('',(0.,-0.25881904510252,0.965925826289068));
#15950=DIRECTION('',(1.,0.,0.));
#15951=DIRECTION('',(0.,0.25881904510252,-0.965925826289068));
#15952=DIRECTION('center_axis',(1.,0.,0.));
#15953=DIRECTION('ref_axis',(0.,0.,-1.));
#15954=DIRECTION('center_axis',(-1.,0.,0.));
#15955=DIRECTION('ref_axis',(0.,1.,0.));
#15956=DIRECTION('center_axis',(1.,0.,0.));
#15957=DIRECTION('ref_axis',(0.,1.,0.));
#15958=DIRECTION('',(0.,-0.25881904510252,0.965925826289069));
#15959=DIRECTION('center_axis',(0.,-0.965925826289069,-0.25881904510252));
#15960=DIRECTION('ref_axis',(0.,0.25881904510252,-0.965925826289069));
#15961=DIRECTION('',(1.,0.,0.));
#15962=DIRECTION('',(-1.,0.,0.));
#15963=DIRECTION('',(0.,0.25881904510252,-0.965925826289069));
#15964=DIRECTION('center_axis',(1.,0.,0.));
#15965=DIRECTION('ref_axis',(0.,0.,-1.));
#15966=DIRECTION('center_axis',(1.,0.,0.));
#15967=DIRECTION('ref_axis',(0.,1.,0.));
#15968=DIRECTION('center_axis',(-1.,0.,0.));
#15969=DIRECTION('ref_axis',(0.,1.,0.));
#15970=DIRECTION('center_axis',(0.,-0.156434465040231,0.987688340595138));
#15971=DIRECTION('ref_axis',(0.,-0.987688340595138,-0.156434465040231));
#15972=DIRECTION('',(-1.,0.,0.));
#15973=DIRECTION('',(0.,0.987688340595138,0.156434465040231));
#15974=DIRECTION('',(1.,0.,0.));
#15975=DIRECTION('',(0.,-0.987688340595138,-0.156434465040231));
#15976=DIRECTION('center_axis',(0.,0.987688340595138,-0.156434465040231));
#15977=DIRECTION('ref_axis',(0.,0.156434465040231,0.987688340595138));
#15978=DIRECTION('',(1.,0.,0.));
#15979=DIRECTION('',(0.,0.156434465040231,0.987688340595138));
#15980=DIRECTION('',(-1.,0.,0.));
#15981=DIRECTION('',(0.,-0.156434465040231,-0.987688340595138));
#15982=DIRECTION('center_axis',(1.,0.,0.));
#15983=DIRECTION('ref_axis',(0.,0.,-1.));
#15984=DIRECTION('center_axis',(1.,0.,0.));
#15985=DIRECTION('ref_axis',(0.,0.,-1.));
#15986=DIRECTION('center_axis',(1.,0.,0.));
#15987=DIRECTION('ref_axis',(0.,0.,-1.));
#15988=DIRECTION('center_axis',(1.,0.,0.));
#15989=DIRECTION('ref_axis',(0.,0.707106781186547,0.707106781186548));
#15990=DIRECTION('center_axis',(1.,0.,0.));
#15991=DIRECTION('ref_axis',(0.,0.,-1.));
#15992=DIRECTION('center_axis',(1.,0.,0.));
#15993=DIRECTION('ref_axis',(0.,0.707106781186547,0.707106781186548));
#15994=DIRECTION('center_axis',(1.,0.,0.));
#15995=DIRECTION('ref_axis',(0.,0.,-1.));
#15996=DIRECTION('center_axis',(-1.,0.,0.));
#15997=DIRECTION('ref_axis',(0.,0.,1.));
#19739=CARTESIAN_POINT('',(0.,0.,0.));
#19740=CARTESIAN_POINT('Origin',(40.9,31.483337699552,36.913331115663));
#19741=CARTESIAN_POINT('',(62.9,30.9136868437562,37.0659686024412));
#19742=CARTESIAN_POINT('',(40.9,30.9136868437562,37.0659686024412));
#19743=CARTESIAN_POINT('',(51.9,30.9136868437562,37.0659686024412));
#19744=CARTESIAN_POINT('',(62.9,28.6606288924974,37.6696736609815));
#19745=CARTESIAN_POINT('',(62.9,28.2957824727981,37.7674339645013));
#19746=CARTESIAN_POINT('',(40.9,28.6606288924974,37.6696736609815));
#19747=CARTESIAN_POINT('',(51.9,28.6606288924974,37.6696736609815));
#19748=CARTESIAN_POINT('',(40.9,28.2957824727981,37.7674339645013));
#19749=CARTESIAN_POINT('Origin',(40.9,29.5660362797969,36.1329752572208));
#19750=CARTESIAN_POINT('',(40.9,30.2666392309999,34.6511540367185));
#19751=CARTESIAN_POINT('Origin',(40.9,22.225,38.1));
#19752=CARTESIAN_POINT('',(40.9,28.0135812797411,35.2548590952589));
#19753=CARTESIAN_POINT('Origin',(40.9,22.225,38.1));
#19754=CARTESIAN_POINT('',(40.9,30.8362900867957,34.4985165499403));
#19755=CARTESIAN_POINT('Origin',(40.9,27.6487348600418,35.3526193987787));
#19756=CARTESIAN_POINT('',(62.9,30.2666392309999,34.6511540367185));
#19757=CARTESIAN_POINT('',(51.9,30.2666392309999,34.6511540367185));
#19758=CARTESIAN_POINT('',(62.9,28.0135812797411,35.2548590952589));
#19759=CARTESIAN_POINT('',(51.9,28.0135812797411,35.2548590952589));
#19760=CARTESIAN_POINT('',(62.9,30.8362900867957,34.4985165499403));
#19761=CARTESIAN_POINT('Origin',(62.9,29.5660362797969,36.1329752572208));
#19762=CARTESIAN_POINT('Origin',(62.9,22.225,38.1));
#19763=CARTESIAN_POINT('Origin',(62.9,22.225,38.1));
#19764=CARTESIAN_POINT('Origin',(40.9,27.8818542494924,45.5246212024587));
#19765=CARTESIAN_POINT('',(62.9,27.4648408804748,45.1076078334411));
#19766=CARTESIAN_POINT('',(40.9,27.4648408804748,45.1076078334411));
#19767=CARTESIAN_POINT('',(51.9,27.4648408804748,45.1076078334411));
#19768=CARTESIAN_POINT('',(62.9,25.8154879877562,43.4582549407226));
#19769=CARTESIAN_POINT('',(62.9,25.5484018715768,43.1911688245431));
#19770=CARTESIAN_POINT('',(40.9,25.8154879877562,43.4582549407226));
#19771=CARTESIAN_POINT('',(51.9,25.8154879877562,43.4582549407226));
#19772=CARTESIAN_POINT('',(40.9,25.5484018715768,43.1911688245431));
#19773=CARTESIAN_POINT('Origin',(40.9,27.5990115370178,43.4740115370178));
#19774=CARTESIAN_POINT('',(40.9,29.2326078334411,43.3398408804748));
#19775=CARTESIAN_POINT('Origin',(40.9,22.225,38.1));
#19776=CARTESIAN_POINT('',(40.9,27.5832549407226,41.6904879877562));
#19777=CARTESIAN_POINT('Origin',(40.9,22.225,38.1));
#19778=CARTESIAN_POINT('',(40.9,29.6496212024587,43.7568542494924));
#19779=CARTESIAN_POINT('Origin',(40.9,27.3161688245431,41.4234018715768));
#19780=CARTESIAN_POINT('',(62.9,29.2326078334411,43.3398408804748));
#19781=CARTESIAN_POINT('',(51.9,29.2326078334411,43.3398408804748));
#19782=CARTESIAN_POINT('',(62.9,27.5832549407226,41.6904879877562));
#19783=CARTESIAN_POINT('',(51.9,27.5832549407226,41.6904879877562));
#19784=CARTESIAN_POINT('',(62.9,29.6496212024587,43.7568542494924));
#19785=CARTESIAN_POINT('Origin',(62.9,27.5990115370178,43.4740115370178));
#19786=CARTESIAN_POINT('Origin',(62.9,22.225,38.1));
#19787=CARTESIAN_POINT('Origin',(62.9,22.225,38.1));
#19788=CARTESIAN_POINT('Origin',(40.9,18.6235165499403,46.7112900867957));
#19789=CARTESIAN_POINT('',(62.9,18.7761540367185,46.1416392309999));
#19790=CARTESIAN_POINT('',(40.9,18.7761540367185,46.1416392309999));
#19791=CARTESIAN_POINT('',(51.9,18.7761540367185,46.1416392309999));
#19792=CARTESIAN_POINT('',(62.9,19.3798590952589,43.8885812797411));
#19793=CARTESIAN_POINT('',(62.9,19.4776193987787,43.5237348600418));
#19794=CARTESIAN_POINT('',(40.9,19.3798590952589,43.8885812797411));
#19795=CARTESIAN_POINT('',(51.9,19.3798590952589,43.8885812797411));
#19796=CARTESIAN_POINT('',(40.9,19.4776193987787,43.5237348600418));
#19797=CARTESIAN_POINT('Origin',(40.9,20.2579752572208,45.4410362797969));
#19798=CARTESIAN_POINT('',(40.9,21.1909686024412,46.7886868437562));
#19799=CARTESIAN_POINT('Origin',(40.9,22.225,38.1));
#19800=CARTESIAN_POINT('',(40.9,21.7946736609815,44.5356288924974));
#19801=CARTESIAN_POINT('Origin',(40.9,22.225,38.1));
#19802=CARTESIAN_POINT('',(40.9,21.038331115663,47.358337699552));
#19803=CARTESIAN_POINT('Origin',(40.9,21.8924339645013,44.1707824727981));
#19804=CARTESIAN_POINT('',(62.9,21.1909686024412,46.7886868437562));
#19805=CARTESIAN_POINT('',(51.9,21.1909686024412,46.7886868437562));
#19806=CARTESIAN_POINT('',(62.9,21.7946736609815,44.5356288924974));
#19807=CARTESIAN_POINT('',(51.9,21.7946736609815,44.5356288924974));
#19808=CARTESIAN_POINT('',(62.9,21.038331115663,47.358337699552));
#19809=CARTESIAN_POINT('Origin',(62.9,20.2579752572208,45.4410362797969));
#19810=CARTESIAN_POINT('Origin',(62.9,22.225,38.1));
#19811=CARTESIAN_POINT('Origin',(62.9,22.225,38.1));
#19812=CARTESIAN_POINT('Origin',(40.9,12.966662300448,39.286668884337));
#19813=CARTESIAN_POINT('',(62.9,13.5363131562438,39.1340313975588));
#19814=CARTESIAN_POINT('',(40.9,13.5363131562438,39.1340313975588));
#19815=CARTESIAN_POINT('',(51.9,13.5363131562438,39.1340313975588));
#19816=CARTESIAN_POINT('',(62.9,15.7893711075026,38.5303263390185));
#19817=CARTESIAN_POINT('',(62.9,16.1542175272019,38.4325660354987));
#19818=CARTESIAN_POINT('',(40.9,15.7893711075026,38.5303263390185));
#19819=CARTESIAN_POINT('',(51.9,15.7893711075026,38.5303263390185));
#19820=CARTESIAN_POINT('',(40.9,16.1542175272019,38.4325660354987));
#19821=CARTESIAN_POINT('Origin',(40.9,14.8839637202031,40.0670247427792));
#19822=CARTESIAN_POINT('',(40.9,14.1833607690001,41.5488459632815));
#19823=CARTESIAN_POINT('Origin',(40.9,22.225,38.1));
#19824=CARTESIAN_POINT('',(40.9,16.4364187202589,40.9451409047411));
#19825=CARTESIAN_POINT('Origin',(40.9,22.225,38.1));
#19826=CARTESIAN_POINT('',(40.9,13.6137099132043,41.7014834500596));
#19827=CARTESIAN_POINT('Origin',(40.9,16.8012651399582,40.8473806012213));
#19828=CARTESIAN_POINT('',(62.9,14.1833607690001,41.5488459632815));
#19829=CARTESIAN_POINT('',(51.9,14.1833607690001,41.5488459632815));
#19830=CARTESIAN_POINT('',(62.9,16.4364187202589,40.9451409047411));
#19831=CARTESIAN_POINT('',(51.9,16.4364187202589,40.9451409047411));
#19832=CARTESIAN_POINT('',(62.9,13.6137099132043,41.7014834500596));
#19833=CARTESIAN_POINT('Origin',(62.9,14.8839637202031,40.0670247427792));
#19834=CARTESIAN_POINT('Origin',(62.9,22.225,38.1));
#19835=CARTESIAN_POINT('Origin',(62.9,22.225,38.1));
#19836=CARTESIAN_POINT('Origin',(40.9,25.8264834500596,29.4887099132043));
#19837=CARTESIAN_POINT('',(62.9,25.6738459632815,30.0583607690001));
#19838=CARTESIAN_POINT('',(40.9,25.6738459632815,30.0583607690001));
#19839=CARTESIAN_POINT('',(51.9,25.6738459632815,30.0583607690001));
#19840=CARTESIAN_POINT('',(62.9,25.0701409047411,32.3114187202589));
#19841=CARTESIAN_POINT('',(62.9,24.9723806012213,32.6762651399582));
#19842=CARTESIAN_POINT('',(40.9,25.0701409047411,32.3114187202589));
#19843=CARTESIAN_POINT('',(51.9,25.0701409047411,32.3114187202589));
#19844=CARTESIAN_POINT('',(40.9,24.9723806012213,32.6762651399582));
#19845=CARTESIAN_POINT('Origin',(40.9,24.1920247427792,30.7589637202031));
#19846=CARTESIAN_POINT('',(40.9,23.2590313975588,29.4113131562438));
#19847=CARTESIAN_POINT('Origin',(40.9,22.225,38.1));
#19848=CARTESIAN_POINT('',(40.9,22.6553263390185,31.6643711075026));
#19849=CARTESIAN_POINT('Origin',(40.9,22.225,38.1));
#19850=CARTESIAN_POINT('',(40.9,23.411668884337,28.841662300448));
#19851=CARTESIAN_POINT('Origin',(40.9,22.5575660354987,32.0292175272019));
#19852=CARTESIAN_POINT('',(62.9,23.2590313975588,29.4113131562438));
#19853=CARTESIAN_POINT('',(51.9,23.2590313975588,29.4113131562438));
#19854=CARTESIAN_POINT('',(62.9,22.6553263390185,31.6643711075026));
#19855=CARTESIAN_POINT('',(51.9,22.6553263390185,31.6643711075026));
#19856=CARTESIAN_POINT('',(62.9,23.411668884337,28.841662300448));
#19857=CARTESIAN_POINT('Origin',(62.9,24.1920247427792,30.7589637202031));
#19858=CARTESIAN_POINT('Origin',(62.9,22.225,38.1));
#19859=CARTESIAN_POINT('Origin',(62.9,22.225,38.1));
#19860=CARTESIAN_POINT('Origin',(32.85,22.225,38.1));
#19861=CARTESIAN_POINT('',(70.65,15.8544102031614,37.0909977004905));
#19862=CARTESIAN_POINT('',(33.15,15.8544102031614,37.0909977004905));
#19863=CARTESIAN_POINT('',(51.9,15.8544102031614,37.0909977004905));
#19864=CARTESIAN_POINT('',(70.65,13.5827270197925,36.731198430898));
#19865=CARTESIAN_POINT('',(70.65,25.3710786325259,38.5982899034296));
#19866=CARTESIAN_POINT('',(33.15,13.5827270197925,36.731198430898));
#19867=CARTESIAN_POINT('',(51.9,13.5827270197925,36.731198430898));
#19868=CARTESIAN_POINT('',(33.15,26.4929361293956,38.7759746751952));
#19869=CARTESIAN_POINT('Origin',(32.85,20.5433295008175,27.4823503386023));
#19870=CARTESIAN_POINT('',(33.15,21.2159977004905,31.7294102031614));
#19871=CARTESIAN_POINT('',(70.65,21.2159977004905,31.7294102031614));
#19872=CARTESIAN_POINT('',(51.9,21.2159977004905,31.7294102031614));
#19873=CARTESIAN_POINT('',(33.15,20.856198430898,29.4577270197926));
#19874=CARTESIAN_POINT('',(33.15,21.4912286210131,33.4671498444963));
#19875=CARTESIAN_POINT('',(70.65,20.856198430898,29.4577270197926));
#19876=CARTESIAN_POINT('',(51.9,20.856198430898,29.4577270197926));
#19877=CARTESIAN_POINT('',(70.65,21.4630861178828,33.2894650727307));
#19878=CARTESIAN_POINT('Origin',(70.65,28.675,38.1));
#19879=CARTESIAN_POINT('Origin',(70.65,22.225,38.1));
#19880=CARTESIAN_POINT('Origin',(70.65,22.225,38.1));
#19881=CARTESIAN_POINT('Origin',(51.9,22.225,38.1));
#19882=CARTESIAN_POINT('Origin',(33.15,22.225,38.1));
#19883=CARTESIAN_POINT('Origin',(51.9,22.225,38.1));
#19884=CARTESIAN_POINT('Origin',(33.15,22.225,38.1));
#19885=CARTESIAN_POINT('Origin',(33.15,30.975,38.1));
#71778=UNCERTAINTY_MEASURE_WITH_UNIT(LENGTH_MEASURE(0.01),#71796,
'DISTANCE_ACCURACY_VALUE',
'Maximum model space distance between geometric entities at asserted c
onnectivities');
#71783=UNCERTAINTY_MEASURE_WITH_UNIT(LENGTH_MEASURE(0.01),#71796,
'DISTANCE_ACCURACY_VALUE',
'Maximum model space distance between geometric entities at asserted c
onnectivities');
#71790=(
GEOMETRIC_REPRESENTATION_CONTEXT(3)
GLOBAL_UNCERTAINTY_ASSIGNED_CONTEXT((#71778))
GLOBAL_UNIT_ASSIGNED_CONTEXT((#71796,#71798,#71799))
REPRESENTATION_CONTEXT('','3D')
);
#71795=(
GEOMETRIC_REPRESENTATION_CONTEXT(3)
GLOBAL_UNCERTAINTY_ASSIGNED_CONTEXT((#71783))
GLOBAL_UNIT_ASSIGNED_CONTEXT((#71796,#71798,#71799))
REPRESENTATION_CONTEXT('','3D')
);
#71796=(
LENGTH_UNIT()
NAMED_UNIT(*)
SI_UNIT(.MILLI.,.METRE.)
);
#71798=(
NAMED_UNIT(*)
PLANE_ANGLE_UNIT()
SI_UNIT($,.RADIAN.)
);
#71799=(
NAMED_UNIT(*)
SI_UNIT($,.STERADIAN.)
SOLID_ANGLE_UNIT()
);
#71806=SHAPE_DEFINITION_REPRESENTATION(#71817,#72022);
#71817=PRODUCT_DEFINITION_SHAPE('',$,#72034);
#72022=SHAPE_REPRESENTATION('',(#14060),#71790);
#72027=PRODUCT_DEFINITION_CONTEXT('part definition',#72062,'design');
#72034=PRODUCT_DEFINITION('Super Smart Ball Retainer',
'Super Smart Ball Retainer',#72045,#72027);
#72045=PRODUCT_DEFINITION_FORMATION('',$,#72070);
#72062=APPLICATION_CONTEXT(
'Core Data for Automotive Mechanical Design Process');
#72063=PRODUCT_CONTEXT('part definition',#72062,'mechanical');
#72070=PRODUCT('Super Smart Ball Retainer','Super Smart Ball Retainer',
$,(#72063));
#72081=PRESENTATION_STYLE_ASSIGNMENT((#72092));
#72092=SURFACE_STYLE_USAGE(.BOTH.,#72103);
#72103=SURFACE_SIDE_STYLE('',(#72114));
#72114=SURFACE_STYLE_FILL_AREA(#72125);
#72125=FILL_AREA_STYLE('Opaque(70,72,76)',(#72136));
#72136=FILL_AREA_STYLE_COLOUR('Opaque(70,72,76)',#72147);
#72147=COLOUR_RGB('Opaque(70,72,76)', 0.08235294, 0.09019608, 0.10196078);
ENDSEC;
END-ISO-10303-21;
